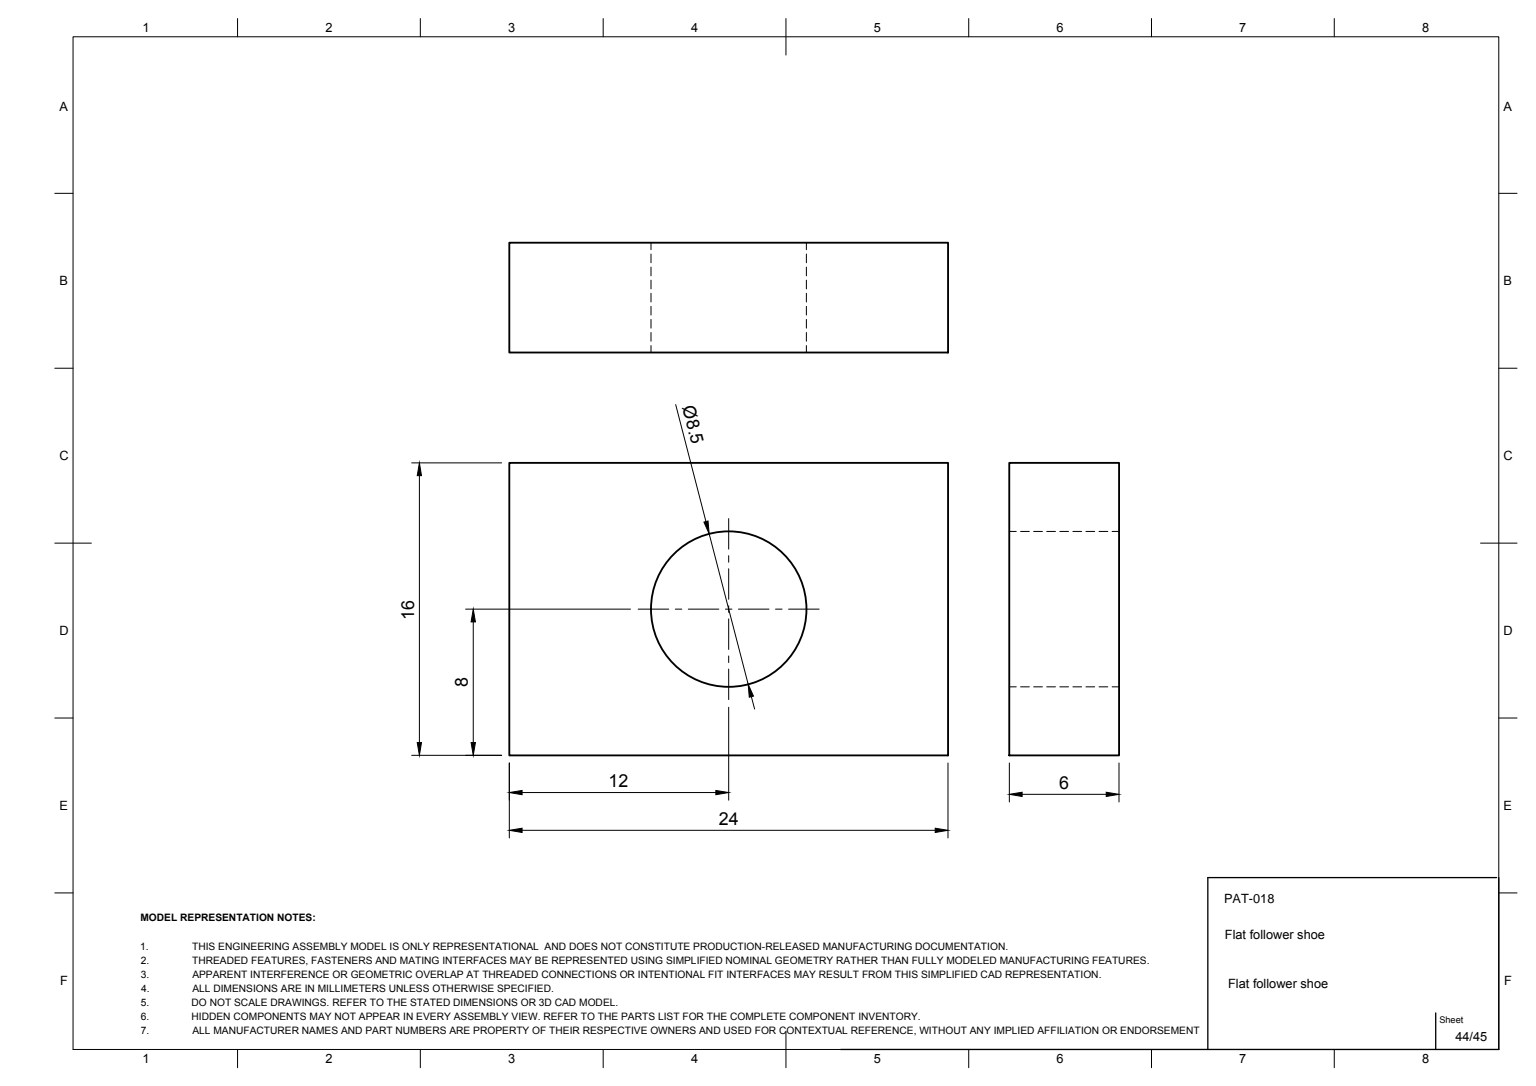
ISO-10303-21;
HEADER;
/* Generated by software containing ST-Developer
 * from STEP Tools, Inc. (www.steptools.com) 
 */

FILE_DESCRIPTION(
/* description */ ('Cam-driven reciprocating slide'),
/* implementation_level */ '2;1');

FILE_NAME(
/* name */ 'Flat follower shoe.step',
/* time_stamp */ '2026-10-28T03:25:20-07:00',
/* author */ (''),
/* organization */ (''),
/* preprocessor_version */ 'ST-DEVELOPER v20.2',
/* originating_system */ 'Autodesk Translation Framework v15.17.0.0',
/* authorisation */ '');

FILE_SCHEMA (('AUTOMOTIVE_DESIGN { 1 0 10303 214 3 1 1 }'));
ENDSEC;

DATA;
#10=MECHANICAL_DESIGN_GEOMETRIC_PRESENTATION_REPRESENTATION('',(#463),#13277);
#382=SHAPE_REPRESENTATION_RELATIONSHIP('SRR','None',#13479,#419);
#419=ADVANCED_BREP_SHAPE_REPRESENTATION('',(#504),#13274);
#463=STYLED_ITEM('',(#13706),#504);
#504=MANIFOLD_SOLID_BREP('Body1',#6442);
#667=FACE_BOUND('',#1800,.T.);
#668=FACE_BOUND('',#1802,.T.);
#885=PLANE('',#7621);
#886=PLANE('',#7622);
#887=PLANE('',#7623);
#888=PLANE('',#7624);
#889=PLANE('',#7625);
#890=PLANE('',#7626);
#1255=FACE_OUTER_BOUND('',#1794,.T.);
#1256=FACE_OUTER_BOUND('',#1795,.T.);
#1257=FACE_OUTER_BOUND('',#1796,.T.);
#1258=FACE_OUTER_BOUND('',#1797,.T.);
#1259=FACE_OUTER_BOUND('',#1798,.T.);
#1260=FACE_OUTER_BOUND('',#1799,.T.);
#1261=FACE_OUTER_BOUND('',#1801,.T.);
#1794=EDGE_LOOP('',(#5790,#5791,#5792,#5793));
#1795=EDGE_LOOP('',(#5794,#5795,#5796,#5797));
#1796=EDGE_LOOP('',(#5798,#5799,#5800,#5801));
#1797=EDGE_LOOP('',(#5802,#5803,#5804,#5805));
#1798=EDGE_LOOP('',(#5806,#5807,#5808,#5809));
#1799=EDGE_LOOP('',(#5810,#5811,#5812,#5813));
#1800=EDGE_LOOP('',(#5814));
#1801=EDGE_LOOP('',(#5815,#5816,#5817,#5818));
#1802=EDGE_LOOP('',(#5819));
#2239=LINE('',#13076,#2678);
#2240=LINE('',#13081,#2679);
#2241=LINE('',#13083,#2680);
#2242=LINE('',#13085,#2681);
#2243=LINE('',#13086,#2682);
#2244=LINE('',#13089,#2683);
#2245=LINE('',#13091,#2684);
#2246=LINE('',#13092,#2685);
#2247=LINE('',#13095,#2686);
#2248=LINE('',#13097,#2687);
#2249=LINE('',#13098,#2688);
#2250=LINE('',#13100,#2689);
#2251=LINE('',#13101,#2690);
#2678=VECTOR('',#9609,0.425);
#2679=VECTOR('',#9614,1.);
#2680=VECTOR('',#9615,1.);
#2681=VECTOR('',#9616,1.);
#2682=VECTOR('',#9617,1.);
#2683=VECTOR('',#9620,1.);
#2684=VECTOR('',#9621,1.);
#2685=VECTOR('',#9622,1.);
#2686=VECTOR('',#9625,1.);
#2687=VECTOR('',#9626,1.);
#2688=VECTOR('',#9627,1.);
#2689=VECTOR('',#9630,1.);
#2690=VECTOR('',#9631,1.);
#3017=CIRCLE('',#7619,0.425);
#3018=CIRCLE('',#7620,0.425);
#3524=VERTEX_POINT('',#13073);
#3525=VERTEX_POINT('',#13075);
#3526=VERTEX_POINT('',#13079);
#3527=VERTEX_POINT('',#13080);
#3528=VERTEX_POINT('',#13082);
#3529=VERTEX_POINT('',#13084);
#3530=VERTEX_POINT('',#13088);
#3531=VERTEX_POINT('',#13090);
#3532=VERTEX_POINT('',#13094);
#3533=VERTEX_POINT('',#13096);
#4285=EDGE_CURVE('',#3524,#3524,#3017,.T.);
#4286=EDGE_CURVE('',#3524,#3525,#2239,.T.);
#4287=EDGE_CURVE('',#3525,#3525,#3018,.T.);
#4288=EDGE_CURVE('',#3526,#3527,#2240,.T.);
#4289=EDGE_CURVE('',#3527,#3528,#2241,.T.);
#4290=EDGE_CURVE('',#3529,#3528,#2242,.T.);
#4291=EDGE_CURVE('',#3526,#3529,#2243,.T.);
#4292=EDGE_CURVE('',#3530,#3526,#2244,.T.);
#4293=EDGE_CURVE('',#3531,#3529,#2245,.T.);
#4294=EDGE_CURVE('',#3530,#3531,#2246,.T.);
#4295=EDGE_CURVE('',#3532,#3530,#2247,.T.);
#4296=EDGE_CURVE('',#3533,#3531,#2248,.T.);
#4297=EDGE_CURVE('',#3532,#3533,#2249,.T.);
#4298=EDGE_CURVE('',#3527,#3532,#2250,.T.);
#4299=EDGE_CURVE('',#3528,#3533,#2251,.T.);
#5790=ORIENTED_EDGE('',*,*,#4285,.F.);
#5791=ORIENTED_EDGE('',*,*,#4286,.T.);
#5792=ORIENTED_EDGE('',*,*,#4287,.F.);
#5793=ORIENTED_EDGE('',*,*,#4286,.F.);
#5794=ORIENTED_EDGE('',*,*,#4288,.T.);
#5795=ORIENTED_EDGE('',*,*,#4289,.T.);
#5796=ORIENTED_EDGE('',*,*,#4290,.F.);
#5797=ORIENTED_EDGE('',*,*,#4291,.F.);
#5798=ORIENTED_EDGE('',*,*,#4292,.T.);
#5799=ORIENTED_EDGE('',*,*,#4291,.T.);
#5800=ORIENTED_EDGE('',*,*,#4293,.F.);
#5801=ORIENTED_EDGE('',*,*,#4294,.F.);
#5802=ORIENTED_EDGE('',*,*,#4295,.T.);
#5803=ORIENTED_EDGE('',*,*,#4294,.T.);
#5804=ORIENTED_EDGE('',*,*,#4296,.F.);
#5805=ORIENTED_EDGE('',*,*,#4297,.F.);
#5806=ORIENTED_EDGE('',*,*,#4298,.T.);
#5807=ORIENTED_EDGE('',*,*,#4297,.T.);
#5808=ORIENTED_EDGE('',*,*,#4299,.F.);
#5809=ORIENTED_EDGE('',*,*,#4289,.F.);
#5810=ORIENTED_EDGE('',*,*,#4299,.T.);
#5811=ORIENTED_EDGE('',*,*,#4296,.T.);
#5812=ORIENTED_EDGE('',*,*,#4293,.T.);
#5813=ORIENTED_EDGE('',*,*,#4290,.T.);
#5814=ORIENTED_EDGE('',*,*,#4287,.T.);
#5815=ORIENTED_EDGE('',*,*,#4298,.F.);
#5816=ORIENTED_EDGE('',*,*,#4288,.F.);
#5817=ORIENTED_EDGE('',*,*,#4292,.F.);
#5818=ORIENTED_EDGE('',*,*,#4295,.F.);
#5819=ORIENTED_EDGE('',*,*,#4285,.T.);
#6010=CYLINDRICAL_SURFACE('',#7618,0.425);
#6373=ADVANCED_FACE('',(#1255),#6010,.F.);
#6374=ADVANCED_FACE('',(#1256),#885,.T.);
#6375=ADVANCED_FACE('',(#1257),#886,.T.);
#6376=ADVANCED_FACE('',(#1258),#887,.T.);
#6377=ADVANCED_FACE('',(#1259),#888,.T.);
#6378=ADVANCED_FACE('',(#1260,#667),#889,.T.);
#6379=ADVANCED_FACE('',(#1261,#668),#890,.F.);
#6442=CLOSED_SHELL('',(#6373,#6374,#6375,#6376,#6377,#6378,#6379));
#7617=AXIS2_PLACEMENT_3D('',#13071,#9603,#9604);
#7618=AXIS2_PLACEMENT_3D('',#13072,#9605,#9606);
#7619=AXIS2_PLACEMENT_3D('',#13074,#9607,#9608);
#7620=AXIS2_PLACEMENT_3D('',#13077,#9610,#9611);
#7621=AXIS2_PLACEMENT_3D('',#13078,#9612,#9613);
#7622=AXIS2_PLACEMENT_3D('',#13087,#9618,#9619);
#7623=AXIS2_PLACEMENT_3D('',#13093,#9623,#9624);
#7624=AXIS2_PLACEMENT_3D('',#13099,#9628,#9629);
#7625=AXIS2_PLACEMENT_3D('',#13102,#9632,#9633);
#7626=AXIS2_PLACEMENT_3D('',#13103,#9634,#9635);
#9603=DIRECTION('axis',(0.,0.,1.));
#9604=DIRECTION('refdir',(1.,0.,0.));
#9605=DIRECTION('center_axis',(0.,0.,1.));
#9606=DIRECTION('ref_axis',(1.,0.,0.));
#9607=DIRECTION('center_axis',(0.,0.,1.));
#9608=DIRECTION('ref_axis',(1.,0.,0.));
#9609=DIRECTION('',(0.,0.,1.));
#9610=DIRECTION('center_axis',(0.,0.,-1.));
#9611=DIRECTION('ref_axis',(1.,0.,0.));
#9612=DIRECTION('center_axis',(0.,1.,0.));
#9613=DIRECTION('ref_axis',(-1.,0.,0.));
#9614=DIRECTION('',(-1.,0.,0.));
#9615=DIRECTION('',(0.,0.,1.));
#9616=DIRECTION('',(-1.,0.,0.));
#9617=DIRECTION('',(0.,0.,1.));
#9618=DIRECTION('center_axis',(1.,0.,0.));
#9619=DIRECTION('ref_axis',(0.,1.,0.));
#9620=DIRECTION('',(0.,1.,0.));
#9621=DIRECTION('',(0.,1.,0.));
#9622=DIRECTION('',(0.,0.,1.));
#9623=DIRECTION('center_axis',(0.,-1.,0.));
#9624=DIRECTION('ref_axis',(1.,0.,0.));
#9625=DIRECTION('',(1.,0.,0.));
#9626=DIRECTION('',(1.,0.,0.));
#9627=DIRECTION('',(0.,0.,1.));
#9628=DIRECTION('center_axis',(-1.,0.,0.));
#9629=DIRECTION('ref_axis',(0.,-1.,0.));
#9630=DIRECTION('',(0.,-1.,0.));
#9631=DIRECTION('',(0.,-1.,0.));
#9632=DIRECTION('center_axis',(0.,0.,1.));
#9633=DIRECTION('ref_axis',(1.,0.,0.));
#9634=DIRECTION('center_axis',(0.,0.,1.));
#9635=DIRECTION('ref_axis',(1.,0.,0.));
#13071=CARTESIAN_POINT('',(0.,0.,0.));
#13072=CARTESIAN_POINT('Origin',(0.,0.,6.9));
#13073=CARTESIAN_POINT('',(-0.425,-5.20474889637625E-17,7.));
#13074=CARTESIAN_POINT('Origin',(0.,0.,7.));
#13075=CARTESIAN_POINT('',(-0.425,5.20474889637625E-17,7.6));
#13076=CARTESIAN_POINT('',(-0.425,-5.20474889637625E-17,6.9));
#13077=CARTESIAN_POINT('Origin',(0.,0.,7.6));
#13078=CARTESIAN_POINT('Origin',(1.2,0.8,7.));
#13079=CARTESIAN_POINT('',(1.2,0.8,7.));
#13080=CARTESIAN_POINT('',(-1.2,0.8,7.));
#13081=CARTESIAN_POINT('',(1.2,0.8,7.));
#13082=CARTESIAN_POINT('',(-1.2,0.8,7.6));
#13083=CARTESIAN_POINT('',(-1.2,0.8,7.));
#13084=CARTESIAN_POINT('',(1.2,0.8,7.6));
#13085=CARTESIAN_POINT('',(1.2,0.8,7.6));
#13086=CARTESIAN_POINT('',(1.2,0.8,7.));
#13087=CARTESIAN_POINT('Origin',(1.2,-0.8,7.));
#13088=CARTESIAN_POINT('',(1.2,-0.8,7.));
#13089=CARTESIAN_POINT('',(1.2,-0.8,7.));
#13090=CARTESIAN_POINT('',(1.2,-0.8,7.6));
#13091=CARTESIAN_POINT('',(1.2,-0.8,7.6));
#13092=CARTESIAN_POINT('',(1.2,-0.8,7.));
#13093=CARTESIAN_POINT('Origin',(-1.2,-0.8,7.));
#13094=CARTESIAN_POINT('',(-1.2,-0.8,7.));
#13095=CARTESIAN_POINT('',(-1.2,-0.8,7.));
#13096=CARTESIAN_POINT('',(-1.2,-0.8,7.6));
#13097=CARTESIAN_POINT('',(-1.2,-0.8,7.6));
#13098=CARTESIAN_POINT('',(-1.2,-0.8,7.));
#13099=CARTESIAN_POINT('Origin',(-1.2,0.8,7.));
#13100=CARTESIAN_POINT('',(-1.2,0.8,7.));
#13101=CARTESIAN_POINT('',(-1.2,0.8,7.6));
#13102=CARTESIAN_POINT('Origin',(0.,0.,7.6));
#13103=CARTESIAN_POINT('Origin',(0.,0.,7.));
#13230=UNCERTAINTY_MEASURE_WITH_UNIT(LENGTH_MEASURE(0.001),#13278,
'DISTANCE_ACCURACY_VALUE',
'Maximum model space distance between geometric entities at asserted c
onnectivities');
#13233=UNCERTAINTY_MEASURE_WITH_UNIT(LENGTH_MEASURE(0.001),#13278,
'DISTANCE_ACCURACY_VALUE',
'Maximum model space distance between geometric entities at asserted c
onnectivities');
#13274=(
GEOMETRIC_REPRESENTATION_CONTEXT(3)
GLOBAL_UNCERTAINTY_ASSIGNED_CONTEXT((#13230))
GLOBAL_UNIT_ASSIGNED_CONTEXT((#13278,#13280,#13281))
REPRESENTATION_CONTEXT('','3D')
);
#13277=(
GEOMETRIC_REPRESENTATION_CONTEXT(3)
GLOBAL_UNCERTAINTY_ASSIGNED_CONTEXT((#13233))
GLOBAL_UNIT_ASSIGNED_CONTEXT((#13278,#13280,#13281))
REPRESENTATION_CONTEXT('','3D')
);
#13278=(
LENGTH_UNIT()
NAMED_UNIT(*)
SI_UNIT(.CENTI.,.METRE.)
);
#13280=(
NAMED_UNIT(*)
PLANE_ANGLE_UNIT()
SI_UNIT($,.RADIAN.)
);
#13281=(
NAMED_UNIT(*)
SI_UNIT($,.STERADIAN.)
SOLID_ANGLE_UNIT()
);
#13322=SHAPE_DEFINITION_REPRESENTATION(#13430,#13479);
#13430=PRODUCT_DEFINITION_SHAPE('',$,#13523);
#13479=SHAPE_REPRESENTATION('',(#7617),#13274);
#13482=PRODUCT_DEFINITION_CONTEXT('part definition',#13613,'design');
#13523=PRODUCT_DEFINITION('Flat follower shoe','Flat follower shoe',#13566,
#13482);
#13566=PRODUCT_DEFINITION_FORMATION('',$,#13655);
#13613=APPLICATION_CONTEXT(
'Core Data for Automotive Mechanical Design Process');
#13614=PRODUCT_CONTEXT('part definition',#13613,'mechanical');
#13655=PRODUCT('Flat follower shoe','Flat follower shoe',
'Flat follower shoe',(#13614));
#13700=COLOUR_RGB('Light Blue',0.38,0.62,0.78);
#13701=FILL_AREA_STYLE_COLOUR('',#13700);
#13702=FILL_AREA_STYLE('',(#13701));
#13703=SURFACE_STYLE_FILL_AREA(#13702);
#13704=SURFACE_SIDE_STYLE('',(#13703));
#13705=SURFACE_STYLE_USAGE(.BOTH.,#13704);
#13706=PRESENTATION_STYLE_ASSIGNMENT((#13705));
ENDSEC;
END-ISO-10303-21;
